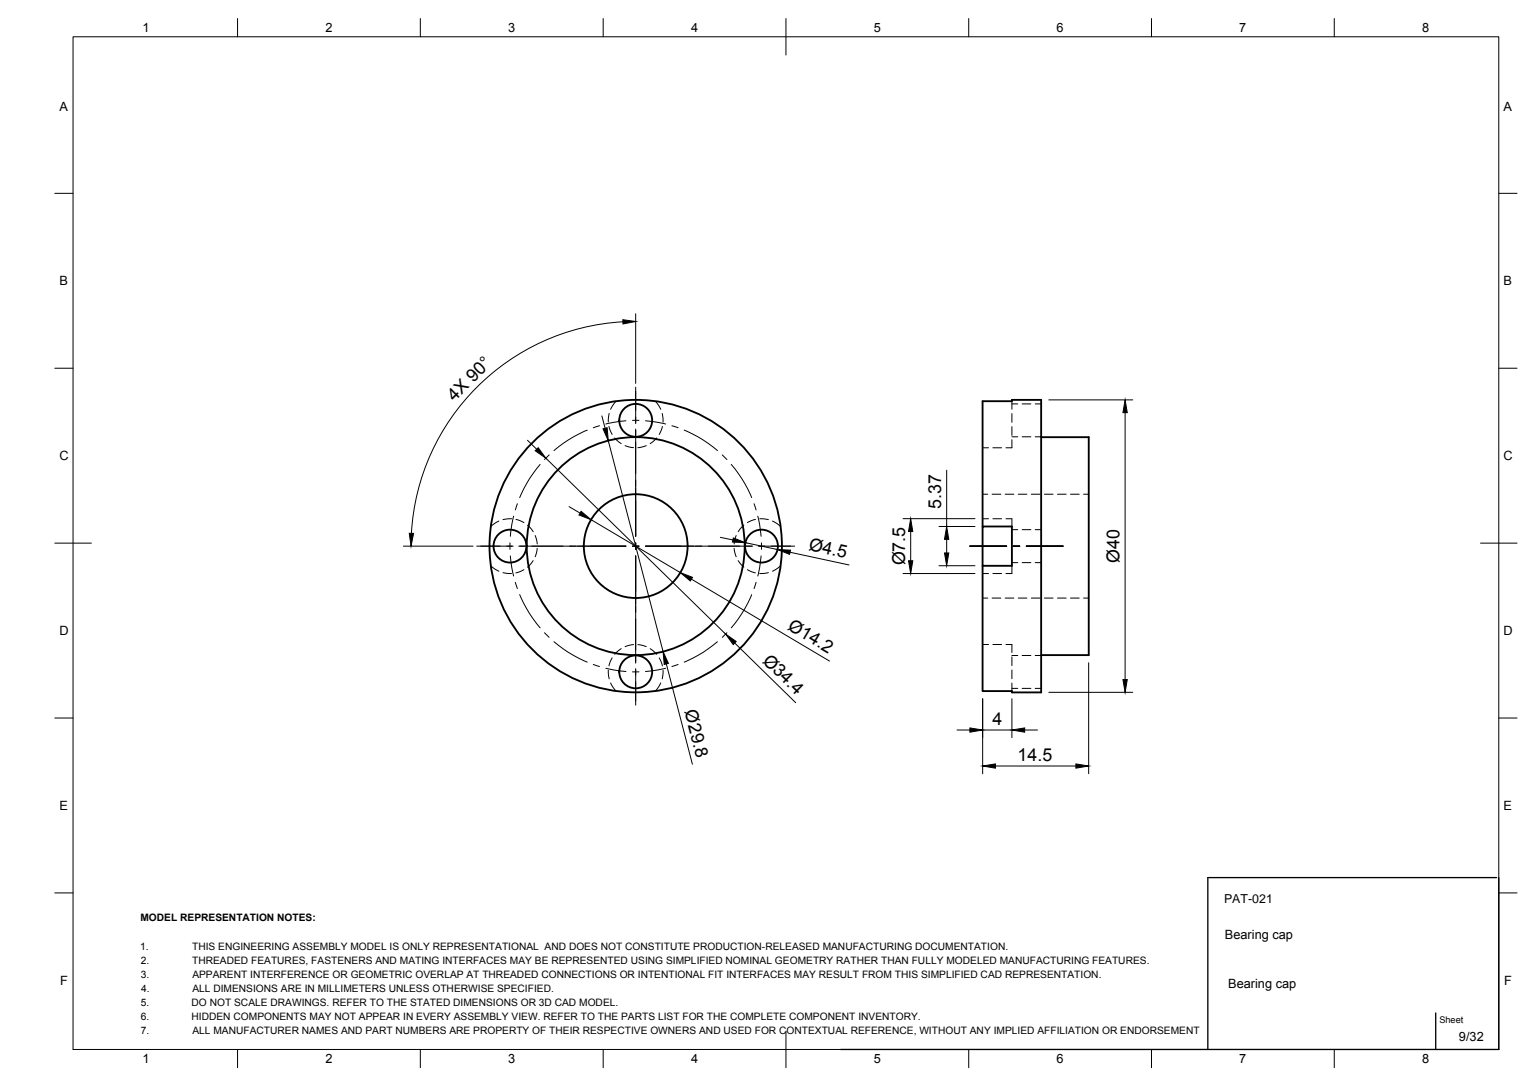
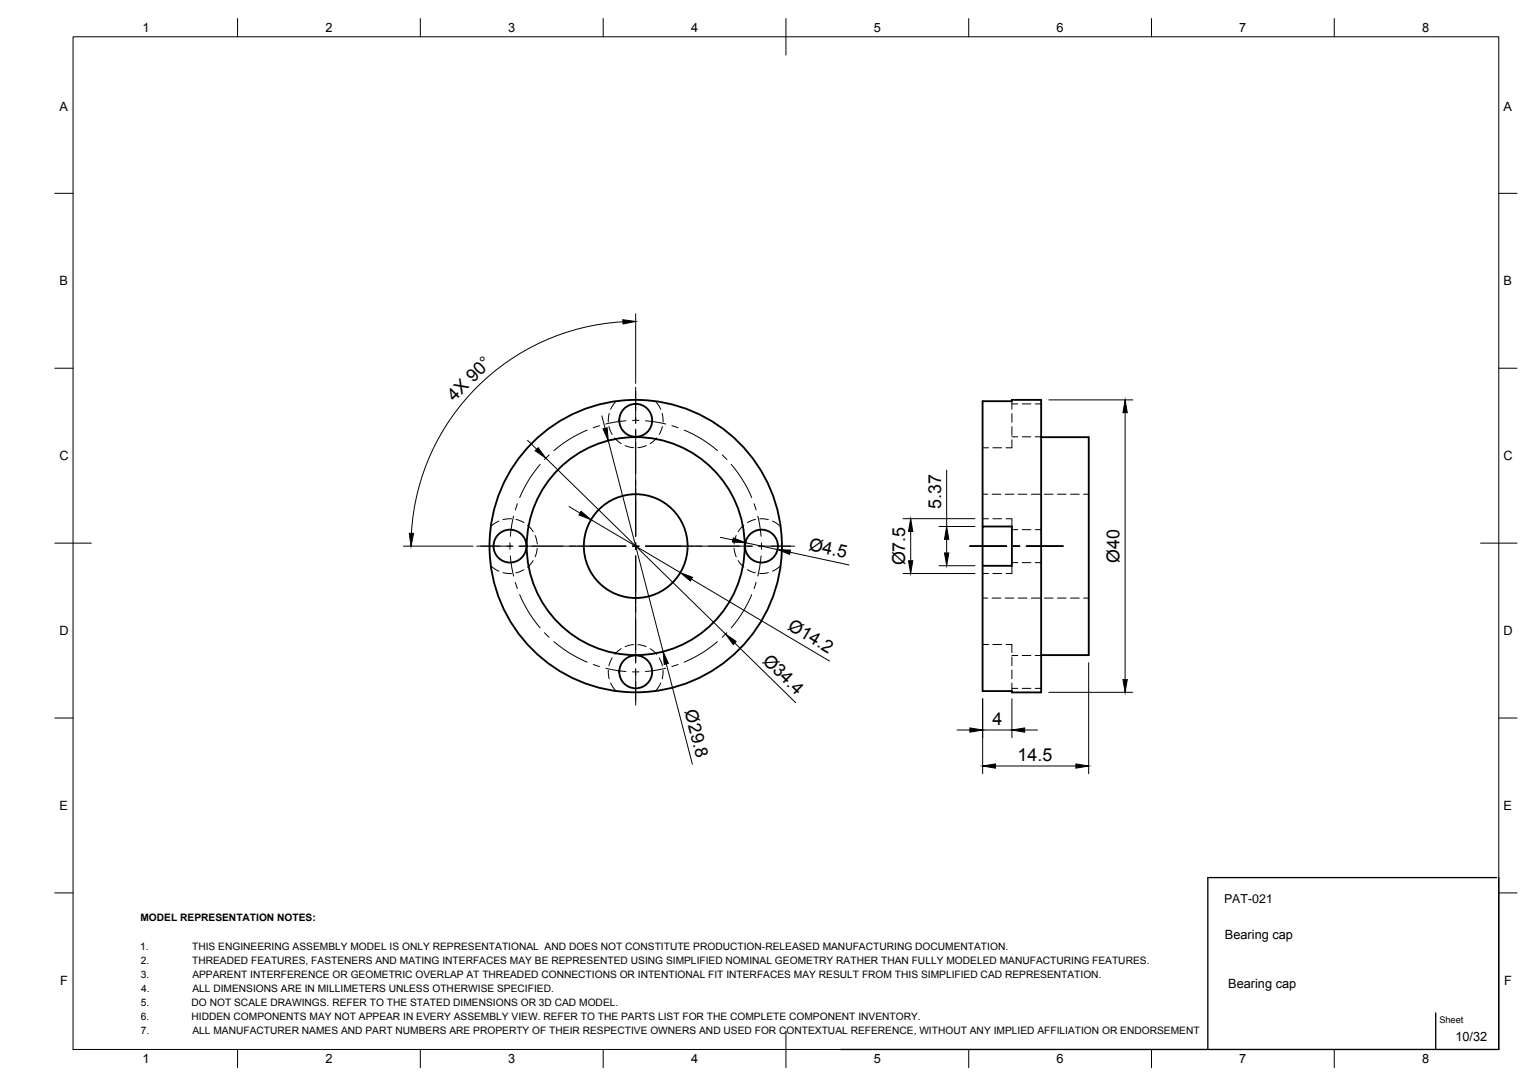
ISO-10303-21;
HEADER;
/* Generated by software containing ST-Developer
 * from STEP Tools, Inc. (www.steptools.com) 
 */

FILE_DESCRIPTION(
/* description */ ('Chain-less indexing wheel (Geneva) drive'),
/* implementation_level */ '2;1');

FILE_NAME(
/* name */ 'Bearing cap.step',
/* time_stamp */ '2026-10-28T03:25:22-07:00',
/* author */ (''),
/* organization */ (''),
/* preprocessor_version */ 'ST-DEVELOPER v20.2',
/* originating_system */ 'Autodesk Translation Framework v15.17.0.0',
/* authorisation */ '');

FILE_SCHEMA (('AUTOMOTIVE_DESIGN { 1 0 10303 214 3 1 1 }'));
ENDSEC;

DATA;
#10=MECHANICAL_DESIGN_GEOMETRIC_PRESENTATION_REPRESENTATION('',(#307),#10957);
#257=SHAPE_REPRESENTATION_RELATIONSHIP('SRR','None',#11070,#282);
#282=ADVANCED_BREP_SHAPE_REPRESENTATION('',(#340),#10933);
#307=STYLED_ITEM('',(#11287),#340);
#340=MANIFOLD_SOLID_BREP('Body1',#5703);
#401=FACE_BOUND('',#1093,.T.);
#402=FACE_BOUND('',#1095,.T.);
#403=FACE_BOUND('',#1098,.T.);
#404=FACE_BOUND('',#1101,.T.);
#405=FACE_BOUND('',#1104,.T.);
#406=FACE_BOUND('',#1111,.T.);
#407=FACE_BOUND('',#1115,.T.);
#408=FACE_BOUND('',#1116,.T.);
#409=FACE_BOUND('',#1117,.T.);
#410=FACE_BOUND('',#1118,.T.);
#411=FACE_BOUND('',#1119,.T.);
#514=PLANE('',#6150);
#515=PLANE('',#6154);
#516=PLANE('',#6160);
#517=PLANE('',#6166);
#518=PLANE('',#6172);
#519=PLANE('',#6189);
#520=PLANE('',#6194);
#724=FACE_OUTER_BOUND('',#1091,.T.);
#725=FACE_OUTER_BOUND('',#1092,.T.);
#726=FACE_OUTER_BOUND('',#1094,.T.);
#727=FACE_OUTER_BOUND('',#1096,.T.);
#728=FACE_OUTER_BOUND('',#1097,.T.);
#729=FACE_OUTER_BOUND('',#1099,.T.);
#730=FACE_OUTER_BOUND('',#1100,.T.);
#731=FACE_OUTER_BOUND('',#1102,.T.);
#732=FACE_OUTER_BOUND('',#1103,.T.);
#733=FACE_OUTER_BOUND('',#1105,.T.);
#734=FACE_OUTER_BOUND('',#1106,.T.);
#735=FACE_OUTER_BOUND('',#1107,.T.);
#736=FACE_OUTER_BOUND('',#1108,.T.);
#737=FACE_OUTER_BOUND('',#1109,.T.);
#738=FACE_OUTER_BOUND('',#1110,.T.);
#739=FACE_OUTER_BOUND('',#1112,.T.);
#740=FACE_OUTER_BOUND('',#1113,.T.);
#741=FACE_OUTER_BOUND('',#1114,.T.);
#1091=EDGE_LOOP('',(#4055,#4056,#4057,#4058));
#1092=EDGE_LOOP('',(#4059,#4060,#4061));
#1093=EDGE_LOOP('',(#4062));
#1094=EDGE_LOOP('',(#4063,#4064));
#1095=EDGE_LOOP('',(#4065));
#1096=EDGE_LOOP('',(#4066,#4067,#4068,#4069));
#1097=EDGE_LOOP('',(#4070,#4071));
#1098=EDGE_LOOP('',(#4072));
#1099=EDGE_LOOP('',(#4073,#4074,#4075,#4076));
#1100=EDGE_LOOP('',(#4077,#4078));
#1101=EDGE_LOOP('',(#4079));
#1102=EDGE_LOOP('',(#4080,#4081,#4082,#4083));
#1103=EDGE_LOOP('',(#4084,#4085,#4086,#4087,#4088,#4089,#4090,#4091));
#1104=EDGE_LOOP('',(#4092));
#1105=EDGE_LOOP('',(#4093,#4094,#4095,#4096));
#1106=EDGE_LOOP('',(#4097,#4098,#4099,#4100));
#1107=EDGE_LOOP('',(#4101,#4102,#4103,#4104));
#1108=EDGE_LOOP('',(#4105,#4106,#4107,#4108));
#1109=EDGE_LOOP('',(#4109,#4110,#4111,#4112));
#1110=EDGE_LOOP('',(#4113));
#1111=EDGE_LOOP('',(#4114));
#1112=EDGE_LOOP('',(#4115,#4116,#4117,#4118));
#1113=EDGE_LOOP('',(#4119,#4120,#4121,#4122,#4123,#4124,#4125,#4126,#4127,
#4128,#4129,#4130,#4131,#4132,#4133,#4134,#4135,#4136,#4137,#4138));
#1114=EDGE_LOOP('',(#4139));
#1115=EDGE_LOOP('',(#4140));
#1116=EDGE_LOOP('',(#4141));
#1117=EDGE_LOOP('',(#4142));
#1118=EDGE_LOOP('',(#4143));
#1119=EDGE_LOOP('',(#4144));
#1517=LINE('',#8995,#1891);
#1518=LINE('',#8999,#1892);
#1519=LINE('',#9016,#1893);
#1520=LINE('',#9019,#1894);
#1521=LINE('',#9029,#1895);
#1522=LINE('',#9032,#1896);
#1523=LINE('',#9042,#1897);
#1524=LINE('',#9045,#1898);
#1525=LINE('',#9056,#1899);
#1526=LINE('',#9060,#1900);
#1527=LINE('',#9064,#1901);
#1528=LINE('',#9068,#1902);
#1529=LINE('',#9073,#1903);
#1530=LINE('',#9079,#1904);
#1531=LINE('',#9082,#1905);
#1891=VECTOR('',#7119,1.);
#1892=VECTOR('',#7122,1.);
#1893=VECTOR('',#7143,1.);
#1894=VECTOR('',#7146,1.);
#1895=VECTOR('',#7157,1.);
#1896=VECTOR('',#7160,1.);
#1897=VECTOR('',#7171,1.);
#1898=VECTOR('',#7174,1.);
#1899=VECTOR('',#7191,0.225);
#1900=VECTOR('',#7196,0.225);
#1901=VECTOR('',#7201,0.225);
#1902=VECTOR('',#7206,0.225);
#1903=VECTOR('',#7211,1.49);
#1904=VECTOR('',#7220,0.71);
#1905=VECTOR('',#7223,2.);
#2229=CIRCLE('',#6148,0.375);
#2230=CIRCLE('',#6149,0.375);
#2231=CIRCLE('',#6151,2.);
#2232=CIRCLE('',#6152,2.);
#2233=CIRCLE('',#6153,0.225);
#2234=CIRCLE('',#6155,2.);
#2235=CIRCLE('',#6156,0.375);
#2236=CIRCLE('',#6157,0.225);
#2237=CIRCLE('',#6159,0.375);
#2238=CIRCLE('',#6161,2.);
#2239=CIRCLE('',#6162,0.375);
#2240=CIRCLE('',#6163,0.225);
#2241=CIRCLE('',#6165,0.375);
#2242=CIRCLE('',#6167,2.);
#2243=CIRCLE('',#6168,0.375);
#2244=CIRCLE('',#6169,0.225);
#2245=CIRCLE('',#6171,0.375);
#2246=CIRCLE('',#6173,2.);
#2247=CIRCLE('',#6174,2.);
#2248=CIRCLE('',#6175,2.);
#2249=CIRCLE('',#6176,2.);
#2250=CIRCLE('',#6177,0.71);
#2251=CIRCLE('',#6179,0.225);
#2252=CIRCLE('',#6181,0.225);
#2253=CIRCLE('',#6183,0.225);
#2254=CIRCLE('',#6185,0.225);
#2255=CIRCLE('',#6187,1.49);
#2256=CIRCLE('',#6188,1.49);
#2257=CIRCLE('',#6190,0.71);
#2258=CIRCLE('',#6193,2.);
#2597=VERTEX_POINT('',#8993);
#2598=VERTEX_POINT('',#8994);
#2599=VERTEX_POINT('',#8996);
#2600=VERTEX_POINT('',#8998);
#2601=VERTEX_POINT('',#9002);
#2602=VERTEX_POINT('',#9005);
#2603=VERTEX_POINT('',#9008);
#2604=VERTEX_POINT('',#9009);
#2605=VERTEX_POINT('',#9012);
#2606=VERTEX_POINT('',#9015);
#2607=VERTEX_POINT('',#9017);
#2608=VERTEX_POINT('',#9021);
#2609=VERTEX_POINT('',#9022);
#2610=VERTEX_POINT('',#9025);
#2611=VERTEX_POINT('',#9028);
#2612=VERTEX_POINT('',#9030);
#2613=VERTEX_POINT('',#9034);
#2614=VERTEX_POINT('',#9035);
#2615=VERTEX_POINT('',#9038);
#2616=VERTEX_POINT('',#9041);
#2617=VERTEX_POINT('',#9043);
#2618=VERTEX_POINT('',#9051);
#2619=VERTEX_POINT('',#9054);
#2620=VERTEX_POINT('',#9058);
#2621=VERTEX_POINT('',#9062);
#2622=VERTEX_POINT('',#9066);
#2623=VERTEX_POINT('',#9070);
#2624=VERTEX_POINT('',#9072);
#2625=VERTEX_POINT('',#9076);
#2626=VERTEX_POINT('',#9081);
#3153=EDGE_CURVE('',#2597,#2598,#1517,.T.);
#3154=EDGE_CURVE('',#2599,#2597,#2229,.T.);
#3155=EDGE_CURVE('',#2600,#2599,#1518,.T.);
#3156=EDGE_CURVE('',#2598,#2600,#2230,.T.);
#3157=EDGE_CURVE('',#2599,#2601,#2231,.T.);
#3158=EDGE_CURVE('',#2601,#2597,#2232,.T.);
#3159=EDGE_CURVE('',#2602,#2602,#2233,.T.);
#3160=EDGE_CURVE('',#2603,#2604,#2234,.T.);
#3161=EDGE_CURVE('',#2603,#2604,#2235,.T.);
#3162=EDGE_CURVE('',#2605,#2605,#2236,.T.);
#3163=EDGE_CURVE('',#2606,#2603,#1519,.T.);
#3164=EDGE_CURVE('',#2607,#2606,#2237,.T.);
#3165=EDGE_CURVE('',#2604,#2607,#1520,.T.);
#3166=EDGE_CURVE('',#2608,#2609,#2238,.T.);
#3167=EDGE_CURVE('',#2608,#2609,#2239,.T.);
#3168=EDGE_CURVE('',#2610,#2610,#2240,.T.);
#3169=EDGE_CURVE('',#2611,#2608,#1521,.T.);
#3170=EDGE_CURVE('',#2612,#2611,#2241,.T.);
#3171=EDGE_CURVE('',#2609,#2612,#1522,.T.);
#3172=EDGE_CURVE('',#2613,#2614,#2242,.T.);
#3173=EDGE_CURVE('',#2613,#2614,#2243,.T.);
#3174=EDGE_CURVE('',#2615,#2615,#2244,.T.);
#3175=EDGE_CURVE('',#2616,#2613,#1523,.T.);
#3176=EDGE_CURVE('',#2617,#2616,#2245,.T.);
#3177=EDGE_CURVE('',#2614,#2617,#1524,.T.);
#3178=EDGE_CURVE('',#2600,#2617,#2246,.T.);
#3179=EDGE_CURVE('',#2616,#2612,#2247,.T.);
#3180=EDGE_CURVE('',#2611,#2607,#2248,.T.);
#3181=EDGE_CURVE('',#2606,#2598,#2249,.T.);
#3182=EDGE_CURVE('',#2618,#2618,#2250,.T.);
#3183=EDGE_CURVE('',#2619,#2619,#2251,.T.);
#3184=EDGE_CURVE('',#2619,#2602,#1525,.T.);
#3185=EDGE_CURVE('',#2620,#2620,#2252,.T.);
#3186=EDGE_CURVE('',#2620,#2605,#1526,.T.);
#3187=EDGE_CURVE('',#2621,#2621,#2253,.T.);
#3188=EDGE_CURVE('',#2621,#2610,#1527,.T.);
#3189=EDGE_CURVE('',#2622,#2622,#2254,.T.);
#3190=EDGE_CURVE('',#2622,#2615,#1528,.T.);
#3191=EDGE_CURVE('',#2623,#2623,#2255,.T.);
#3192=EDGE_CURVE('',#2623,#2624,#1529,.T.);
#3193=EDGE_CURVE('',#2624,#2624,#2256,.T.);
#3194=EDGE_CURVE('',#2625,#2625,#2257,.T.);
#3195=EDGE_CURVE('',#2618,#2625,#1530,.T.);
#3196=EDGE_CURVE('',#2601,#2626,#1531,.T.);
#3197=EDGE_CURVE('',#2626,#2626,#2258,.T.);
#4055=ORIENTED_EDGE('',*,*,#3153,.F.);
#4056=ORIENTED_EDGE('',*,*,#3154,.F.);
#4057=ORIENTED_EDGE('',*,*,#3155,.F.);
#4058=ORIENTED_EDGE('',*,*,#3156,.F.);
#4059=ORIENTED_EDGE('',*,*,#3157,.F.);
#4060=ORIENTED_EDGE('',*,*,#3154,.T.);
#4061=ORIENTED_EDGE('',*,*,#3158,.F.);
#4062=ORIENTED_EDGE('',*,*,#3159,.F.);
#4063=ORIENTED_EDGE('',*,*,#3160,.F.);
#4064=ORIENTED_EDGE('',*,*,#3161,.T.);
#4065=ORIENTED_EDGE('',*,*,#3162,.F.);
#4066=ORIENTED_EDGE('',*,*,#3163,.F.);
#4067=ORIENTED_EDGE('',*,*,#3164,.F.);
#4068=ORIENTED_EDGE('',*,*,#3165,.F.);
#4069=ORIENTED_EDGE('',*,*,#3161,.F.);
#4070=ORIENTED_EDGE('',*,*,#3166,.F.);
#4071=ORIENTED_EDGE('',*,*,#3167,.T.);
#4072=ORIENTED_EDGE('',*,*,#3168,.F.);
#4073=ORIENTED_EDGE('',*,*,#3169,.F.);
#4074=ORIENTED_EDGE('',*,*,#3170,.F.);
#4075=ORIENTED_EDGE('',*,*,#3171,.F.);
#4076=ORIENTED_EDGE('',*,*,#3167,.F.);
#4077=ORIENTED_EDGE('',*,*,#3172,.F.);
#4078=ORIENTED_EDGE('',*,*,#3173,.T.);
#4079=ORIENTED_EDGE('',*,*,#3174,.F.);
#4080=ORIENTED_EDGE('',*,*,#3175,.F.);
#4081=ORIENTED_EDGE('',*,*,#3176,.F.);
#4082=ORIENTED_EDGE('',*,*,#3177,.F.);
#4083=ORIENTED_EDGE('',*,*,#3173,.F.);
#4084=ORIENTED_EDGE('',*,*,#3156,.T.);
#4085=ORIENTED_EDGE('',*,*,#3178,.T.);
#4086=ORIENTED_EDGE('',*,*,#3176,.T.);
#4087=ORIENTED_EDGE('',*,*,#3179,.T.);
#4088=ORIENTED_EDGE('',*,*,#3170,.T.);
#4089=ORIENTED_EDGE('',*,*,#3180,.T.);
#4090=ORIENTED_EDGE('',*,*,#3164,.T.);
#4091=ORIENTED_EDGE('',*,*,#3181,.T.);
#4092=ORIENTED_EDGE('',*,*,#3182,.T.);
#4093=ORIENTED_EDGE('',*,*,#3183,.F.);
#4094=ORIENTED_EDGE('',*,*,#3184,.T.);
#4095=ORIENTED_EDGE('',*,*,#3159,.T.);
#4096=ORIENTED_EDGE('',*,*,#3184,.F.);
#4097=ORIENTED_EDGE('',*,*,#3185,.F.);
#4098=ORIENTED_EDGE('',*,*,#3186,.T.);
#4099=ORIENTED_EDGE('',*,*,#3162,.T.);
#4100=ORIENTED_EDGE('',*,*,#3186,.F.);
#4101=ORIENTED_EDGE('',*,*,#3187,.F.);
#4102=ORIENTED_EDGE('',*,*,#3188,.T.);
#4103=ORIENTED_EDGE('',*,*,#3168,.T.);
#4104=ORIENTED_EDGE('',*,*,#3188,.F.);
#4105=ORIENTED_EDGE('',*,*,#3189,.F.);
#4106=ORIENTED_EDGE('',*,*,#3190,.T.);
#4107=ORIENTED_EDGE('',*,*,#3174,.T.);
#4108=ORIENTED_EDGE('',*,*,#3190,.F.);
#4109=ORIENTED_EDGE('',*,*,#3191,.F.);
#4110=ORIENTED_EDGE('',*,*,#3192,.T.);
#4111=ORIENTED_EDGE('',*,*,#3193,.T.);
#4112=ORIENTED_EDGE('',*,*,#3192,.F.);
#4113=ORIENTED_EDGE('',*,*,#3193,.F.);
#4114=ORIENTED_EDGE('',*,*,#3194,.F.);
#4115=ORIENTED_EDGE('',*,*,#3182,.F.);
#4116=ORIENTED_EDGE('',*,*,#3195,.T.);
#4117=ORIENTED_EDGE('',*,*,#3194,.T.);
#4118=ORIENTED_EDGE('',*,*,#3195,.F.);
#4119=ORIENTED_EDGE('',*,*,#3153,.T.);
#4120=ORIENTED_EDGE('',*,*,#3181,.F.);
#4121=ORIENTED_EDGE('',*,*,#3163,.T.);
#4122=ORIENTED_EDGE('',*,*,#3160,.T.);
#4123=ORIENTED_EDGE('',*,*,#3165,.T.);
#4124=ORIENTED_EDGE('',*,*,#3180,.F.);
#4125=ORIENTED_EDGE('',*,*,#3169,.T.);
#4126=ORIENTED_EDGE('',*,*,#3166,.T.);
#4127=ORIENTED_EDGE('',*,*,#3171,.T.);
#4128=ORIENTED_EDGE('',*,*,#3179,.F.);
#4129=ORIENTED_EDGE('',*,*,#3175,.T.);
#4130=ORIENTED_EDGE('',*,*,#3172,.T.);
#4131=ORIENTED_EDGE('',*,*,#3177,.T.);
#4132=ORIENTED_EDGE('',*,*,#3178,.F.);
#4133=ORIENTED_EDGE('',*,*,#3155,.T.);
#4134=ORIENTED_EDGE('',*,*,#3157,.T.);
#4135=ORIENTED_EDGE('',*,*,#3196,.T.);
#4136=ORIENTED_EDGE('',*,*,#3197,.T.);
#4137=ORIENTED_EDGE('',*,*,#3196,.F.);
#4138=ORIENTED_EDGE('',*,*,#3158,.T.);
#4139=ORIENTED_EDGE('',*,*,#3197,.F.);
#4140=ORIENTED_EDGE('',*,*,#3191,.T.);
#4141=ORIENTED_EDGE('',*,*,#3189,.T.);
#4142=ORIENTED_EDGE('',*,*,#3187,.T.);
#4143=ORIENTED_EDGE('',*,*,#3185,.T.);
#4144=ORIENTED_EDGE('',*,*,#3183,.T.);
#5273=CYLINDRICAL_SURFACE('',#6147,0.375);
#5274=CYLINDRICAL_SURFACE('',#6158,0.375);
#5275=CYLINDRICAL_SURFACE('',#6164,0.375);
#5276=CYLINDRICAL_SURFACE('',#6170,0.375);
#5277=CYLINDRICAL_SURFACE('',#6178,0.225);
#5278=CYLINDRICAL_SURFACE('',#6180,0.225);
#5279=CYLINDRICAL_SURFACE('',#6182,0.225);
#5280=CYLINDRICAL_SURFACE('',#6184,0.225);
#5281=CYLINDRICAL_SURFACE('',#6186,1.49);
#5282=CYLINDRICAL_SURFACE('',#6191,0.71);
#5283=CYLINDRICAL_SURFACE('',#6192,2.);
#5438=ADVANCED_FACE('',(#724),#5273,.F.);
#5439=ADVANCED_FACE('',(#725,#401),#514,.T.);
#5440=ADVANCED_FACE('',(#726,#402),#515,.T.);
#5441=ADVANCED_FACE('',(#727),#5274,.F.);
#5442=ADVANCED_FACE('',(#728,#403),#516,.T.);
#5443=ADVANCED_FACE('',(#729),#5275,.F.);
#5444=ADVANCED_FACE('',(#730,#404),#517,.T.);
#5445=ADVANCED_FACE('',(#731),#5276,.F.);
#5446=ADVANCED_FACE('',(#732,#405),#518,.T.);
#5447=ADVANCED_FACE('',(#733),#5277,.F.);
#5448=ADVANCED_FACE('',(#734),#5278,.F.);
#5449=ADVANCED_FACE('',(#735),#5279,.F.);
#5450=ADVANCED_FACE('',(#736),#5280,.F.);
#5451=ADVANCED_FACE('',(#737),#5281,.T.);
#5452=ADVANCED_FACE('',(#738,#406),#519,.F.);
#5453=ADVANCED_FACE('',(#739),#5282,.F.);
#5454=ADVANCED_FACE('',(#740),#5283,.T.);
#5455=ADVANCED_FACE('',(#741,#407,#408,#409,#410,#411),#520,.F.);
#5703=CLOSED_SHELL('',(#5438,#5439,#5440,#5441,#5442,#5443,#5444,#5445,
#5446,#5447,#5448,#5449,#5450,#5451,#5452,#5453,#5454,#5455));
#6146=AXIS2_PLACEMENT_3D('',#8991,#7115,#7116);
#6147=AXIS2_PLACEMENT_3D('',#8992,#7117,#7118);
#6148=AXIS2_PLACEMENT_3D('',#8997,#7120,#7121);
#6149=AXIS2_PLACEMENT_3D('',#9000,#7123,#7124);
#6150=AXIS2_PLACEMENT_3D('',#9001,#7125,#7126);
#6151=AXIS2_PLACEMENT_3D('',#9003,#7127,#7128);
#6152=AXIS2_PLACEMENT_3D('',#9004,#7129,#7130);
#6153=AXIS2_PLACEMENT_3D('',#9006,#7131,#7132);
#6154=AXIS2_PLACEMENT_3D('',#9007,#7133,#7134);
#6155=AXIS2_PLACEMENT_3D('',#9010,#7135,#7136);
#6156=AXIS2_PLACEMENT_3D('',#9011,#7137,#7138);
#6157=AXIS2_PLACEMENT_3D('',#9013,#7139,#7140);
#6158=AXIS2_PLACEMENT_3D('',#9014,#7141,#7142);
#6159=AXIS2_PLACEMENT_3D('',#9018,#7144,#7145);
#6160=AXIS2_PLACEMENT_3D('',#9020,#7147,#7148);
#6161=AXIS2_PLACEMENT_3D('',#9023,#7149,#7150);
#6162=AXIS2_PLACEMENT_3D('',#9024,#7151,#7152);
#6163=AXIS2_PLACEMENT_3D('',#9026,#7153,#7154);
#6164=AXIS2_PLACEMENT_3D('',#9027,#7155,#7156);
#6165=AXIS2_PLACEMENT_3D('',#9031,#7158,#7159);
#6166=AXIS2_PLACEMENT_3D('',#9033,#7161,#7162);
#6167=AXIS2_PLACEMENT_3D('',#9036,#7163,#7164);
#6168=AXIS2_PLACEMENT_3D('',#9037,#7165,#7166);
#6169=AXIS2_PLACEMENT_3D('',#9039,#7167,#7168);
#6170=AXIS2_PLACEMENT_3D('',#9040,#7169,#7170);
#6171=AXIS2_PLACEMENT_3D('',#9044,#7172,#7173);
#6172=AXIS2_PLACEMENT_3D('',#9046,#7175,#7176);
#6173=AXIS2_PLACEMENT_3D('',#9047,#7177,#7178);
#6174=AXIS2_PLACEMENT_3D('',#9048,#7179,#7180);
#6175=AXIS2_PLACEMENT_3D('',#9049,#7181,#7182);
#6176=AXIS2_PLACEMENT_3D('',#9050,#7183,#7184);
#6177=AXIS2_PLACEMENT_3D('',#9052,#7185,#7186);
#6178=AXIS2_PLACEMENT_3D('',#9053,#7187,#7188);
#6179=AXIS2_PLACEMENT_3D('',#9055,#7189,#7190);
#6180=AXIS2_PLACEMENT_3D('',#9057,#7192,#7193);
#6181=AXIS2_PLACEMENT_3D('',#9059,#7194,#7195);
#6182=AXIS2_PLACEMENT_3D('',#9061,#7197,#7198);
#6183=AXIS2_PLACEMENT_3D('',#9063,#7199,#7200);
#6184=AXIS2_PLACEMENT_3D('',#9065,#7202,#7203);
#6185=AXIS2_PLACEMENT_3D('',#9067,#7204,#7205);
#6186=AXIS2_PLACEMENT_3D('',#9069,#7207,#7208);
#6187=AXIS2_PLACEMENT_3D('',#9071,#7209,#7210);
#6188=AXIS2_PLACEMENT_3D('',#9074,#7212,#7213);
#6189=AXIS2_PLACEMENT_3D('',#9075,#7214,#7215);
#6190=AXIS2_PLACEMENT_3D('',#9077,#7216,#7217);
#6191=AXIS2_PLACEMENT_3D('',#9078,#7218,#7219);
#6192=AXIS2_PLACEMENT_3D('',#9080,#7221,#7222);
#6193=AXIS2_PLACEMENT_3D('',#9083,#7224,#7225);
#6194=AXIS2_PLACEMENT_3D('',#9084,#7226,#7227);
#7115=DIRECTION('axis',(0.,0.,1.));
#7116=DIRECTION('refdir',(1.,0.,0.));
#7117=DIRECTION('center_axis',(0.,0.,1.));
#7118=DIRECTION('ref_axis',(1.,0.,0.));
#7119=DIRECTION('',(0.,0.,1.));
#7120=DIRECTION('center_axis',(0.,0.,1.));
#7121=DIRECTION('ref_axis',(1.,0.,0.));
#7122=DIRECTION('',(0.,0.,-1.));
#7123=DIRECTION('center_axis',(0.,0.,-1.));
#7124=DIRECTION('ref_axis',(1.,0.,0.));
#7125=DIRECTION('center_axis',(0.,0.,1.));
#7126=DIRECTION('ref_axis',(1.,0.,0.));
#7127=DIRECTION('center_axis',(0.,0.,-1.));
#7128=DIRECTION('ref_axis',(1.,0.,0.));
#7129=DIRECTION('center_axis',(0.,0.,-1.));
#7130=DIRECTION('ref_axis',(1.,0.,0.));
#7131=DIRECTION('center_axis',(0.,0.,1.));
#7132=DIRECTION('ref_axis',(1.,0.,0.));
#7133=DIRECTION('center_axis',(0.,0.,1.));
#7134=DIRECTION('ref_axis',(1.,0.,0.));
#7135=DIRECTION('center_axis',(0.,0.,-1.));
#7136=DIRECTION('ref_axis',(1.,0.,0.));
#7137=DIRECTION('center_axis',(0.,0.,1.));
#7138=DIRECTION('ref_axis',(1.,0.,0.));
#7139=DIRECTION('center_axis',(0.,0.,1.));
#7140=DIRECTION('ref_axis',(1.,0.,0.));
#7141=DIRECTION('center_axis',(0.,0.,1.));
#7142=DIRECTION('ref_axis',(-1.83697019872103E-16,-1.,0.));
#7143=DIRECTION('',(0.,0.,-1.));
#7144=DIRECTION('center_axis',(0.,0.,-1.));
#7145=DIRECTION('ref_axis',(1.,0.,0.));
#7146=DIRECTION('',(0.,0.,1.));
#7147=DIRECTION('center_axis',(0.,0.,1.));
#7148=DIRECTION('ref_axis',(1.,0.,0.));
#7149=DIRECTION('center_axis',(0.,0.,-1.));
#7150=DIRECTION('ref_axis',(1.,0.,0.));
#7151=DIRECTION('center_axis',(0.,0.,1.));
#7152=DIRECTION('ref_axis',(1.,0.,0.));
#7153=DIRECTION('center_axis',(0.,0.,1.));
#7154=DIRECTION('ref_axis',(1.,0.,0.));
#7155=DIRECTION('center_axis',(0.,0.,1.));
#7156=DIRECTION('ref_axis',(-1.,1.22464679914735E-16,0.));
#7157=DIRECTION('',(0.,0.,-1.));
#7158=DIRECTION('center_axis',(0.,0.,-1.));
#7159=DIRECTION('ref_axis',(1.,0.,0.));
#7160=DIRECTION('',(0.,0.,1.));
#7161=DIRECTION('center_axis',(0.,0.,1.));
#7162=DIRECTION('ref_axis',(1.,0.,0.));
#7163=DIRECTION('center_axis',(0.,0.,-1.));
#7164=DIRECTION('ref_axis',(1.,0.,0.));
#7165=DIRECTION('center_axis',(0.,0.,1.));
#7166=DIRECTION('ref_axis',(1.,0.,0.));
#7167=DIRECTION('center_axis',(0.,0.,1.));
#7168=DIRECTION('ref_axis',(1.,0.,0.));
#7169=DIRECTION('center_axis',(0.,0.,1.));
#7170=DIRECTION('ref_axis',(6.12323399573677E-17,1.,0.));
#7171=DIRECTION('',(0.,0.,-1.));
#7172=DIRECTION('center_axis',(0.,0.,-1.));
#7173=DIRECTION('ref_axis',(1.,0.,0.));
#7174=DIRECTION('',(0.,0.,1.));
#7175=DIRECTION('center_axis',(0.,0.,1.));
#7176=DIRECTION('ref_axis',(1.,0.,0.));
#7177=DIRECTION('center_axis',(0.,0.,1.));
#7178=DIRECTION('ref_axis',(1.,0.,0.));
#7179=DIRECTION('center_axis',(0.,0.,1.));
#7180=DIRECTION('ref_axis',(1.,0.,0.));
#7181=DIRECTION('center_axis',(0.,0.,1.));
#7182=DIRECTION('ref_axis',(1.,0.,0.));
#7183=DIRECTION('center_axis',(0.,0.,1.));
#7184=DIRECTION('ref_axis',(1.,0.,0.));
#7185=DIRECTION('center_axis',(0.,0.,-1.));
#7186=DIRECTION('ref_axis',(1.,0.,0.));
#7187=DIRECTION('center_axis',(0.,0.,1.));
#7188=DIRECTION('ref_axis',(1.,0.,0.));
#7189=DIRECTION('center_axis',(0.,0.,1.));
#7190=DIRECTION('ref_axis',(1.,0.,0.));
#7191=DIRECTION('',(0.,0.,1.));
#7192=DIRECTION('center_axis',(0.,0.,1.));
#7193=DIRECTION('ref_axis',(1.,0.,0.));
#7194=DIRECTION('center_axis',(0.,0.,1.));
#7195=DIRECTION('ref_axis',(1.,0.,0.));
#7196=DIRECTION('',(0.,0.,1.));
#7197=DIRECTION('center_axis',(0.,0.,1.));
#7198=DIRECTION('ref_axis',(1.,0.,0.));
#7199=DIRECTION('center_axis',(0.,0.,1.));
#7200=DIRECTION('ref_axis',(1.,0.,0.));
#7201=DIRECTION('',(0.,0.,1.));
#7202=DIRECTION('center_axis',(0.,0.,1.));
#7203=DIRECTION('ref_axis',(1.,0.,0.));
#7204=DIRECTION('center_axis',(0.,0.,1.));
#7205=DIRECTION('ref_axis',(1.,0.,0.));
#7206=DIRECTION('',(0.,0.,1.));
#7207=DIRECTION('center_axis',(0.,0.,1.));
#7208=DIRECTION('ref_axis',(1.,0.,0.));
#7209=DIRECTION('center_axis',(0.,0.,1.));
#7210=DIRECTION('ref_axis',(1.,0.,0.));
#7211=DIRECTION('',(0.,0.,-1.));
#7212=DIRECTION('center_axis',(0.,0.,1.));
#7213=DIRECTION('ref_axis',(1.,0.,0.));
#7214=DIRECTION('center_axis',(0.,0.,1.));
#7215=DIRECTION('ref_axis',(1.,0.,0.));
#7216=DIRECTION('center_axis',(0.,0.,-1.));
#7217=DIRECTION('ref_axis',(1.,0.,0.));
#7218=DIRECTION('center_axis',(0.,0.,1.));
#7219=DIRECTION('ref_axis',(1.,0.,0.));
#7220=DIRECTION('',(0.,0.,-1.));
#7221=DIRECTION('center_axis',(0.,0.,1.));
#7222=DIRECTION('ref_axis',(1.,0.,0.));
#7223=DIRECTION('',(0.,0.,-1.));
#7224=DIRECTION('center_axis',(0.,0.,1.));
#7225=DIRECTION('ref_axis',(1.,0.,0.));
#7226=DIRECTION('center_axis',(0.,0.,1.));
#7227=DIRECTION('ref_axis',(1.,0.,0.));
#8991=CARTESIAN_POINT('',(0.,0.,0.));
#8992=CARTESIAN_POINT('Origin',(-1.72,2.10639249453345E-16,4.));
#8993=CARTESIAN_POINT('',(-1.9819113372093,0.268379305165721,4.));
#8994=CARTESIAN_POINT('',(-1.9819113372093,0.26837930516572,4.4));
#8995=CARTESIAN_POINT('',(-1.9819113372093,0.268379305165721,4.));
#8996=CARTESIAN_POINT('',(-1.9819113372093,-0.268379305165721,4.));
#8997=CARTESIAN_POINT('Origin',(-1.72,2.10639249453345E-16,4.));
#8998=CARTESIAN_POINT('',(-1.9819113372093,-0.268379305165719,4.4));
#8999=CARTESIAN_POINT('',(-1.9819113372093,-0.268379305165721,4.));
#9000=CARTESIAN_POINT('Origin',(-1.72,2.10639249453345E-16,4.4));
#9001=CARTESIAN_POINT('Origin',(-1.72,2.22044604925031E-16,4.));
#9002=CARTESIAN_POINT('',(-2.,-2.44929359829471E-16,4.));
#9003=CARTESIAN_POINT('Origin',(0.,0.,4.));
#9004=CARTESIAN_POINT('Origin',(0.,0.,4.));
#9005=CARTESIAN_POINT('',(-1.945,1.83084696472529E-16,4.));
#9006=CARTESIAN_POINT('Origin',(-1.72,2.10639249453345E-16,4.));
#9007=CARTESIAN_POINT('Origin',(1.11022302462516E-16,1.72,4.));
#9008=CARTESIAN_POINT('',(-0.268379305165721,1.9819113372093,4.));
#9009=CARTESIAN_POINT('',(0.268379305165721,1.9819113372093,4.));
#9010=CARTESIAN_POINT('Origin',(0.,0.,4.));
#9011=CARTESIAN_POINT('Origin',(1.05319624726672E-16,1.72,4.));
#9012=CARTESIAN_POINT('',(-0.225,1.72,4.));
#9013=CARTESIAN_POINT('Origin',(1.05319624726672E-16,1.72,4.));
#9014=CARTESIAN_POINT('Origin',(1.05319624726672E-16,1.72,4.));
#9015=CARTESIAN_POINT('',(-0.26837930516572,1.9819113372093,4.4));
#9016=CARTESIAN_POINT('',(-0.268379305165721,1.9819113372093,4.));
#9017=CARTESIAN_POINT('',(0.26837930516572,1.9819113372093,4.4));
#9018=CARTESIAN_POINT('Origin',(1.05319624726672E-16,1.72,4.4));
#9019=CARTESIAN_POINT('',(0.268379305165721,1.9819113372093,4.));
#9020=CARTESIAN_POINT('Origin',(1.72,0.,4.));
#9021=CARTESIAN_POINT('',(1.9819113372093,0.268379305165721,4.));
#9022=CARTESIAN_POINT('',(1.9819113372093,-0.268379305165721,4.));
#9023=CARTESIAN_POINT('Origin',(0.,0.,4.));
#9024=CARTESIAN_POINT('Origin',(1.72,0.,4.));
#9025=CARTESIAN_POINT('',(1.495,-2.75545529808155E-17,4.));
#9026=CARTESIAN_POINT('Origin',(1.72,0.,4.));
#9027=CARTESIAN_POINT('Origin',(1.72,0.,4.));
#9028=CARTESIAN_POINT('',(1.9819113372093,0.26837930516572,4.4));
#9029=CARTESIAN_POINT('',(1.9819113372093,0.268379305165721,4.));
#9030=CARTESIAN_POINT('',(1.9819113372093,-0.26837930516572,4.4));
#9031=CARTESIAN_POINT('Origin',(1.72,0.,4.4));
#9032=CARTESIAN_POINT('',(1.9819113372093,-0.268379305165721,4.));
#9033=CARTESIAN_POINT('Origin',(-3.33066907387547E-16,-1.72,4.));
#9034=CARTESIAN_POINT('',(0.26837930516572,-1.9819113372093,4.));
#9035=CARTESIAN_POINT('',(-0.268379305165721,-1.9819113372093,4.));
#9036=CARTESIAN_POINT('Origin',(0.,0.,4.));
#9037=CARTESIAN_POINT('Origin',(-3.15958874180017E-16,-1.72,4.));
#9038=CARTESIAN_POINT('',(-0.225,-1.72,4.));
#9039=CARTESIAN_POINT('Origin',(-3.15958874180017E-16,-1.72,4.));
#9040=CARTESIAN_POINT('Origin',(-3.15958874180017E-16,-1.72,4.));
#9041=CARTESIAN_POINT('',(0.268379305165719,-1.9819113372093,4.4));
#9042=CARTESIAN_POINT('',(0.26837930516572,-1.9819113372093,4.));
#9043=CARTESIAN_POINT('',(-0.26837930516572,-1.9819113372093,4.4));
#9044=CARTESIAN_POINT('Origin',(-3.15958874180017E-16,-1.72,4.4));
#9045=CARTESIAN_POINT('',(-0.268379305165721,-1.9819113372093,4.));
#9046=CARTESIAN_POINT('Origin',(0.,0.,4.4));
#9047=CARTESIAN_POINT('Origin',(0.,0.,4.4));
#9048=CARTESIAN_POINT('Origin',(0.,0.,4.4));
#9049=CARTESIAN_POINT('Origin',(0.,0.,4.4));
#9050=CARTESIAN_POINT('Origin',(0.,0.,4.4));
#9051=CARTESIAN_POINT('',(-0.71,-8.69499227394621E-17,4.4));
#9052=CARTESIAN_POINT('Origin',(0.,0.,4.4));
#9053=CARTESIAN_POINT('Origin',(-1.72,2.10639249453345E-16,3.5));
#9054=CARTESIAN_POINT('',(-1.945,1.83084696472529E-16,3.6));
#9055=CARTESIAN_POINT('Origin',(-1.72,2.10639249453345E-16,3.6));
#9056=CARTESIAN_POINT('',(-1.945,1.83084696472529E-16,3.5));
#9057=CARTESIAN_POINT('Origin',(1.05319624726672E-16,1.72,3.5));
#9058=CARTESIAN_POINT('',(-0.225,1.72,3.6));
#9059=CARTESIAN_POINT('Origin',(1.05319624726672E-16,1.72,3.6));
#9060=CARTESIAN_POINT('',(-0.225,1.72,3.5));
#9061=CARTESIAN_POINT('Origin',(1.72,0.,3.5));
#9062=CARTESIAN_POINT('',(1.495,-2.75545529808155E-17,3.6));
#9063=CARTESIAN_POINT('Origin',(1.72,0.,3.6));
#9064=CARTESIAN_POINT('',(1.495,-2.75545529808155E-17,3.5));
#9065=CARTESIAN_POINT('Origin',(-3.15958874180017E-16,-1.72,3.5));
#9066=CARTESIAN_POINT('',(-0.225,-1.72,3.6));
#9067=CARTESIAN_POINT('Origin',(-3.15958874180017E-16,-1.72,3.6));
#9068=CARTESIAN_POINT('',(-0.225,-1.72,3.5));
#9069=CARTESIAN_POINT('Origin',(0.,0.,2.95));
#9070=CARTESIAN_POINT('',(-1.49,-1.82472373072956E-16,3.6));
#9071=CARTESIAN_POINT('Origin',(0.,0.,3.6));
#9072=CARTESIAN_POINT('',(-1.49,-1.82472373072956E-16,2.95));
#9073=CARTESIAN_POINT('',(-1.49,-1.82472373072956E-16,2.95));
#9074=CARTESIAN_POINT('Origin',(0.,0.,2.95));
#9075=CARTESIAN_POINT('Origin',(0.,0.,2.95));
#9076=CARTESIAN_POINT('',(-0.71,-8.69499227394621E-17,2.95));
#9077=CARTESIAN_POINT('Origin',(0.,0.,2.95));
#9078=CARTESIAN_POINT('Origin',(0.,0.,3.6));
#9079=CARTESIAN_POINT('',(-0.71,-8.69499227394621E-17,3.6));
#9080=CARTESIAN_POINT('Origin',(0.,0.,3.6));
#9081=CARTESIAN_POINT('',(-2.,-2.44929359829471E-16,3.6));
#9082=CARTESIAN_POINT('',(-2.,-2.44929359829471E-16,3.6));
#9083=CARTESIAN_POINT('Origin',(0.,0.,3.6));
#9084=CARTESIAN_POINT('Origin',(0.,0.,3.6));
#10902=UNCERTAINTY_MEASURE_WITH_UNIT(LENGTH_MEASURE(0.001),#10958,
'DISTANCE_ACCURACY_VALUE',
'Maximum model space distance between geometric entities at asserted c
onnectivities');
#10926=UNCERTAINTY_MEASURE_WITH_UNIT(LENGTH_MEASURE(0.001),#10958,
'DISTANCE_ACCURACY_VALUE',
'Maximum model space distance between geometric entities at asserted c
onnectivities');
#10933=(
GEOMETRIC_REPRESENTATION_CONTEXT(3)
GLOBAL_UNCERTAINTY_ASSIGNED_CONTEXT((#10902))
GLOBAL_UNIT_ASSIGNED_CONTEXT((#10958,#10960,#10961))
REPRESENTATION_CONTEXT('','3D')
);
#10957=(
GEOMETRIC_REPRESENTATION_CONTEXT(3)
GLOBAL_UNCERTAINTY_ASSIGNED_CONTEXT((#10926))
GLOBAL_UNIT_ASSIGNED_CONTEXT((#10958,#10960,#10961))
REPRESENTATION_CONTEXT('','3D')
);
#10958=(
LENGTH_UNIT()
NAMED_UNIT(*)
SI_UNIT(.CENTI.,.METRE.)
);
#10960=(
NAMED_UNIT(*)
PLANE_ANGLE_UNIT()
SI_UNIT($,.RADIAN.)
);
#10961=(
NAMED_UNIT(*)
SI_UNIT($,.STERADIAN.)
SOLID_ANGLE_UNIT()
);
#10968=SHAPE_DEFINITION_REPRESENTATION(#10998,#11070);
#10998=PRODUCT_DEFINITION_SHAPE('',$,#11101);
#11070=SHAPE_REPRESENTATION('',(#6146),#10933);
#11094=PRODUCT_DEFINITION_CONTEXT('part definition',#11186,'design');
#11101=PRODUCT_DEFINITION('Bearing cap','Bearing cap',#11131,#11094);
#11131=PRODUCT_DEFINITION_FORMATION('',$,#11194);
#11186=APPLICATION_CONTEXT(
'Core Data for Automotive Mechanical Design Process');
#11187=PRODUCT_CONTEXT('part definition',#11186,'mechanical');
#11194=PRODUCT('Bearing cap','Bearing cap','Bearing cap',(#11187));
#11281=COLOUR_RGB('Grey',0.48,0.52,0.57);
#11282=FILL_AREA_STYLE_COLOUR('',#11281);
#11283=FILL_AREA_STYLE('',(#11282));
#11284=SURFACE_STYLE_FILL_AREA(#11283);
#11285=SURFACE_SIDE_STYLE('',(#11284));
#11286=SURFACE_STYLE_USAGE(.BOTH.,#11285);
#11287=PRESENTATION_STYLE_ASSIGNMENT((#11286));
ENDSEC;
END-ISO-10303-21;
